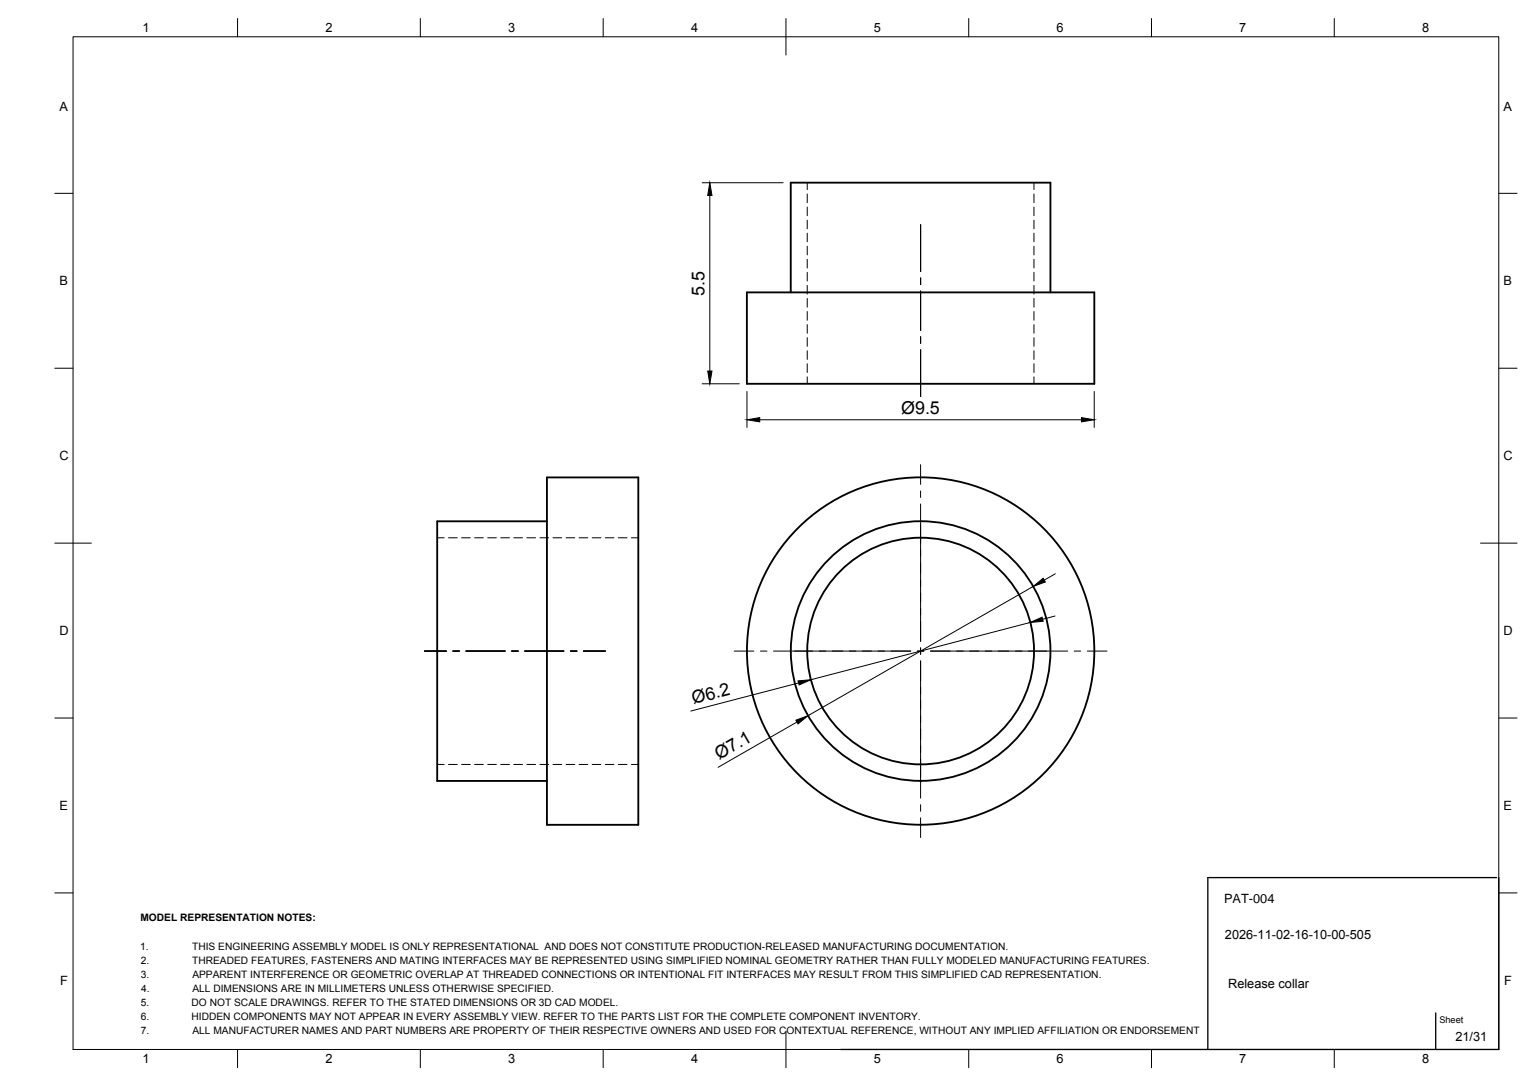
ISO-10303-21;
HEADER;
/* Generated by software containing ST-Developer
 * from STEP Tools, Inc. (www.steptools.com) 
 */

FILE_DESCRIPTION(
/* description */ ('Air blow-off nozzle station'),
/* implementation_level */ '2;1');

FILE_NAME(
/* name */ 'Release collar.step',
/* time_stamp */ '2026-10-27T10:53:54-07:00',
/* author */ (''),
/* organization */ (''),
/* preprocessor_version */ 'ST-DEVELOPER v20.2',
/* originating_system */ 'Autodesk Translation Framework v15.17.0.0',
/* authorisation */ '');

FILE_SCHEMA (('AUTOMOTIVE_DESIGN { 1 0 10303 214 3 1 1 }'));
ENDSEC;

DATA;
#10=MECHANICAL_DESIGN_GEOMETRIC_PRESENTATION_REPRESENTATION('',(#261),#7897);
#211=SHAPE_REPRESENTATION_RELATIONSHIP('SRR','None',#8029,#236);
#236=ADVANCED_BREP_SHAPE_REPRESENTATION('',(#284),#7896);
#261=STYLED_ITEM('',(#8234),#284);
#284=MANIFOLD_SOLID_BREP('Body1',#4312);
#368=FACE_BOUND('',#1130,.T.);
#369=FACE_BOUND('',#1133,.T.);
#370=FACE_BOUND('',#1136,.T.);
#537=PLANE('',#5042);
#538=PLANE('',#5047);
#539=PLANE('',#5051);
#790=FACE_OUTER_BOUND('',#1129,.T.);
#791=FACE_OUTER_BOUND('',#1131,.T.);
#792=FACE_OUTER_BOUND('',#1132,.T.);
#793=FACE_OUTER_BOUND('',#1134,.T.);
#794=FACE_OUTER_BOUND('',#1135,.T.);
#795=FACE_OUTER_BOUND('',#1137,.T.);
#1129=EDGE_LOOP('',(#3941));
#1130=EDGE_LOOP('',(#3942));
#1131=EDGE_LOOP('',(#3943,#3944,#3945,#3946));
#1132=EDGE_LOOP('',(#3947));
#1133=EDGE_LOOP('',(#3948));
#1134=EDGE_LOOP('',(#3949,#3950,#3951,#3952));
#1135=EDGE_LOOP('',(#3953));
#1136=EDGE_LOOP('',(#3954));
#1137=EDGE_LOOP('',(#3955,#3956,#3957,#3958));
#1489=LINE('',#7803,#1843);
#1490=LINE('',#7810,#1844);
#1491=LINE('',#7815,#1845);
#1843=VECTOR('',#6339,0.475);
#1844=VECTOR('',#6348,0.355);
#1845=VECTOR('',#6355,0.31);
#2001=CIRCLE('',#5043,0.475);
#2002=CIRCLE('',#5044,0.31);
#2003=CIRCLE('',#5046,0.475);
#2004=CIRCLE('',#5048,0.355);
#2005=CIRCLE('',#5050,0.355);
#2006=CIRCLE('',#5052,0.31);
#2360=VERTEX_POINT('',#7796);
#2361=VERTEX_POINT('',#7798);
#2362=VERTEX_POINT('',#7801);
#2363=VERTEX_POINT('',#7805);
#2364=VERTEX_POINT('',#7808);
#2365=VERTEX_POINT('',#7812);
#2888=EDGE_CURVE('',#2360,#2360,#2001,.T.);
#2889=EDGE_CURVE('',#2361,#2361,#2002,.T.);
#2890=EDGE_CURVE('',#2362,#2362,#2003,.T.);
#2891=EDGE_CURVE('',#2362,#2360,#1489,.T.);
#2892=EDGE_CURVE('',#2363,#2363,#2004,.T.);
#2893=EDGE_CURVE('',#2364,#2364,#2005,.T.);
#2894=EDGE_CURVE('',#2364,#2363,#1490,.T.);
#2895=EDGE_CURVE('',#2365,#2365,#2006,.T.);
#2896=EDGE_CURVE('',#2365,#2361,#1491,.T.);
#3941=ORIENTED_EDGE('',*,*,#2888,.F.);
#3942=ORIENTED_EDGE('',*,*,#2889,.T.);
#3943=ORIENTED_EDGE('',*,*,#2890,.F.);
#3944=ORIENTED_EDGE('',*,*,#2891,.T.);
#3945=ORIENTED_EDGE('',*,*,#2888,.T.);
#3946=ORIENTED_EDGE('',*,*,#2891,.F.);
#3947=ORIENTED_EDGE('',*,*,#2890,.T.);
#3948=ORIENTED_EDGE('',*,*,#2892,.F.);
#3949=ORIENTED_EDGE('',*,*,#2893,.F.);
#3950=ORIENTED_EDGE('',*,*,#2894,.T.);
#3951=ORIENTED_EDGE('',*,*,#2892,.T.);
#3952=ORIENTED_EDGE('',*,*,#2894,.F.);
#3953=ORIENTED_EDGE('',*,*,#2893,.T.);
#3954=ORIENTED_EDGE('',*,*,#2895,.F.);
#3955=ORIENTED_EDGE('',*,*,#2895,.T.);
#3956=ORIENTED_EDGE('',*,*,#2896,.T.);
#3957=ORIENTED_EDGE('',*,*,#2889,.F.);
#3958=ORIENTED_EDGE('',*,*,#2896,.F.);
#4027=CYLINDRICAL_SURFACE('',#5045,0.475);
#4028=CYLINDRICAL_SURFACE('',#5049,0.355);
#4029=CYLINDRICAL_SURFACE('',#5053,0.31);
#4280=ADVANCED_FACE('',(#790,#368),#537,.T.);
#4281=ADVANCED_FACE('',(#791),#4027,.T.);
#4282=ADVANCED_FACE('',(#792,#369),#538,.T.);
#4283=ADVANCED_FACE('',(#793),#4028,.T.);
#4284=ADVANCED_FACE('',(#794,#370),#539,.T.);
#4285=ADVANCED_FACE('',(#795),#4029,.F.);
#4312=CLOSED_SHELL('',(#4280,#4281,#4282,#4283,#4284,#4285));
#5041=AXIS2_PLACEMENT_3D('',#7794,#6327,#6328);
#5042=AXIS2_PLACEMENT_3D('',#7795,#6329,#6330);
#5043=AXIS2_PLACEMENT_3D('',#7797,#6331,#6332);
#5044=AXIS2_PLACEMENT_3D('',#7799,#6333,#6334);
#5045=AXIS2_PLACEMENT_3D('',#7800,#6335,#6336);
#5046=AXIS2_PLACEMENT_3D('',#7802,#6337,#6338);
#5047=AXIS2_PLACEMENT_3D('',#7804,#6340,#6341);
#5048=AXIS2_PLACEMENT_3D('',#7806,#6342,#6343);
#5049=AXIS2_PLACEMENT_3D('',#7807,#6344,#6345);
#5050=AXIS2_PLACEMENT_3D('',#7809,#6346,#6347);
#5051=AXIS2_PLACEMENT_3D('',#7811,#6349,#6350);
#5052=AXIS2_PLACEMENT_3D('',#7813,#6351,#6352);
#5053=AXIS2_PLACEMENT_3D('',#7814,#6353,#6354);
#6327=DIRECTION('axis',(0.,0.,1.));
#6328=DIRECTION('refdir',(1.,0.,0.));
#6329=DIRECTION('center_axis',(0.,1.,0.));
#6330=DIRECTION('ref_axis',(0.,0.,1.));
#6331=DIRECTION('center_axis',(0.,-1.,0.));
#6332=DIRECTION('ref_axis',(1.,0.,0.));
#6333=DIRECTION('center_axis',(0.,-1.,0.));
#6334=DIRECTION('ref_axis',(1.,0.,0.));
#6335=DIRECTION('center_axis',(0.,-1.,0.));
#6336=DIRECTION('ref_axis',(1.,0.,0.));
#6337=DIRECTION('center_axis',(0.,-1.,0.));
#6338=DIRECTION('ref_axis',(1.,0.,0.));
#6339=DIRECTION('',(0.,1.,0.));
#6340=DIRECTION('center_axis',(0.,-1.,0.));
#6341=DIRECTION('ref_axis',(0.,0.,-1.));
#6342=DIRECTION('center_axis',(0.,-1.,0.));
#6343=DIRECTION('ref_axis',(1.,0.,0.));
#6344=DIRECTION('center_axis',(0.,-1.,0.));
#6345=DIRECTION('ref_axis',(1.,0.,0.));
#6346=DIRECTION('center_axis',(0.,-1.,0.));
#6347=DIRECTION('ref_axis',(1.,0.,0.));
#6348=DIRECTION('',(0.,1.,0.));
#6349=DIRECTION('center_axis',(0.,-1.,0.));
#6350=DIRECTION('ref_axis',(0.,0.,-1.));
#6351=DIRECTION('center_axis',(0.,-1.,0.));
#6352=DIRECTION('ref_axis',(1.,0.,0.));
#6353=DIRECTION('center_axis',(0.,-1.,0.));
#6354=DIRECTION('ref_axis',(1.,0.,0.));
#6355=DIRECTION('',(0.,1.,0.));
#7794=CARTESIAN_POINT('',(0.,0.,0.));
#7795=CARTESIAN_POINT('Origin',(0.475,1.95,0.));
#7796=CARTESIAN_POINT('',(-0.475,1.95,-5.81707229594993E-17));
#7797=CARTESIAN_POINT('Origin',(0.,1.95,0.));
#7798=CARTESIAN_POINT('',(-0.31,1.95,-3.7964050773568E-17));
#7799=CARTESIAN_POINT('Origin',(0.,1.95,0.));
#7800=CARTESIAN_POINT('Origin',(0.,1.825,0.));
#7801=CARTESIAN_POINT('',(-0.475,1.7,-5.81707229594993E-17));
#7802=CARTESIAN_POINT('Origin',(0.,1.7,0.));
#7803=CARTESIAN_POINT('',(-0.475,1.825,-5.81707229594993E-17));
#7804=CARTESIAN_POINT('Origin',(0.355,1.7,0.));
#7805=CARTESIAN_POINT('',(-0.355,1.7,-4.3474961369731E-17));
#7806=CARTESIAN_POINT('Origin',(0.,1.7,0.));
#7807=CARTESIAN_POINT('Origin',(0.,1.55,0.));
#7808=CARTESIAN_POINT('',(-0.355,1.4,-4.3474961369731E-17));
#7809=CARTESIAN_POINT('Origin',(0.,1.4,0.));
#7810=CARTESIAN_POINT('',(-0.355,1.55,-4.3474961369731E-17));
#7811=CARTESIAN_POINT('Origin',(0.31,1.4,0.));
#7812=CARTESIAN_POINT('',(-0.31,1.4,-3.7964050773568E-17));
#7813=CARTESIAN_POINT('Origin',(0.,1.4,0.));
#7814=CARTESIAN_POINT('Origin',(0.,1.675,0.));
#7815=CARTESIAN_POINT('',(-0.31,1.675,-3.7964050773568E-17));
#7864=UNCERTAINTY_MEASURE_WITH_UNIT(LENGTH_MEASURE(0.001),#7898,
'DISTANCE_ACCURACY_VALUE',
'Maximum model space distance between geometric entities at asserted c
onnectivities');
#7865=UNCERTAINTY_MEASURE_WITH_UNIT(LENGTH_MEASURE(0.001),#7898,
'DISTANCE_ACCURACY_VALUE',
'Maximum model space distance between geometric entities at asserted c
onnectivities');
#7896=(
GEOMETRIC_REPRESENTATION_CONTEXT(3)
GLOBAL_UNCERTAINTY_ASSIGNED_CONTEXT((#7864))
GLOBAL_UNIT_ASSIGNED_CONTEXT((#7898,#7900,#7901))
REPRESENTATION_CONTEXT('','3D')
);
#7897=(
GEOMETRIC_REPRESENTATION_CONTEXT(3)
GLOBAL_UNCERTAINTY_ASSIGNED_CONTEXT((#7865))
GLOBAL_UNIT_ASSIGNED_CONTEXT((#7898,#7900,#7901))
REPRESENTATION_CONTEXT('','3D')
);
#7898=(
LENGTH_UNIT()
NAMED_UNIT(*)
SI_UNIT(.CENTI.,.METRE.)
);
#7900=(
NAMED_UNIT(*)
PLANE_ANGLE_UNIT()
SI_UNIT($,.RADIAN.)
);
#7901=(
NAMED_UNIT(*)
SI_UNIT($,.STERADIAN.)
SOLID_ANGLE_UNIT()
);
#7932=SHAPE_DEFINITION_REPRESENTATION(#7980,#8029);
#7980=PRODUCT_DEFINITION_SHAPE('',$,#8061);
#8029=SHAPE_REPRESENTATION('',(#5041),#7896);
#8030=PRODUCT_DEFINITION_CONTEXT('part definition',#8125,'design');
#8061=PRODUCT_DEFINITION('Release collar','Release collar',#8092,#8030);
#8092=PRODUCT_DEFINITION_FORMATION('',$,#8157);
#8125=APPLICATION_CONTEXT(
'Core Data for Automotive Mechanical Design Process');
#8126=PRODUCT_CONTEXT('part definition',#8125,'mechanical');
#8157=PRODUCT('Release collar','Release collar','Release collar',(#8126));
#8228=COLOUR_RGB('Off White',0.89,0.88,0.83);
#8229=FILL_AREA_STYLE_COLOUR('',#8228);
#8230=FILL_AREA_STYLE('',(#8229));
#8231=SURFACE_STYLE_FILL_AREA(#8230);
#8232=SURFACE_SIDE_STYLE('',(#8231));
#8233=SURFACE_STYLE_USAGE(.BOTH.,#8232);
#8234=PRESENTATION_STYLE_ASSIGNMENT((#8233));
ENDSEC;
END-ISO-10303-21;
